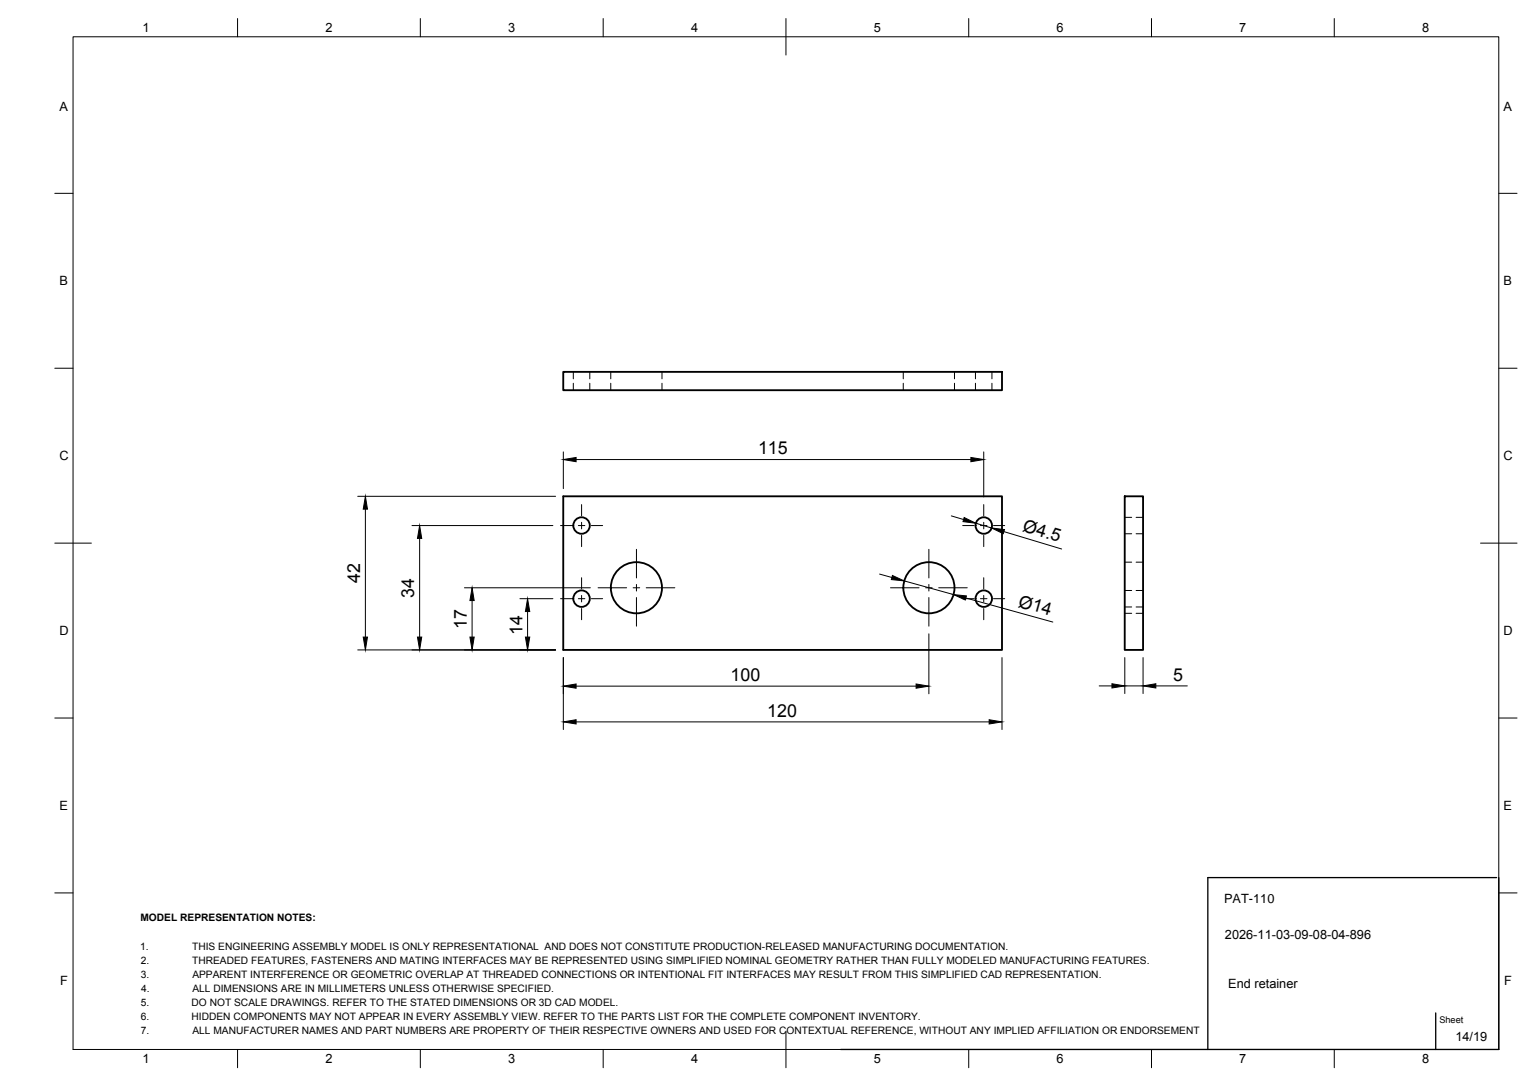
ISO-10303-21;
HEADER;
/* Generated by software containing ST-Developer
 * from STEP Tools, Inc. (www.steptools.com) 
 */

FILE_DESCRIPTION(
/* description */ ('Twin-shaft manual slide'),
/* implementation_level */ '2;1');

FILE_NAME(
/* name */ 'End retainer.step',
/* time_stamp */ '2026-10-27T18:38:08-07:00',
/* author */ (''),
/* organization */ (''),
/* preprocessor_version */ 'ST-DEVELOPER v20.2',
/* originating_system */ 'Autodesk Translation Framework v15.17.0.0',
/* authorisation */ '');

FILE_SCHEMA (('AUTOMOTIVE_DESIGN { 1 0 10303 214 3 1 1 }'));
ENDSEC;

DATA;
#10=MECHANICAL_DESIGN_GEOMETRIC_PRESENTATION_REPRESENTATION('',(#286),#6463);
#254=SHAPE_REPRESENTATION_RELATIONSHIP('SRR','None',#6574,#270);
#270=ADVANCED_BREP_SHAPE_REPRESENTATION('',(#301),#6457);
#286=STYLED_ITEM('',(#6726),#301);
#301=MANIFOLD_SOLID_BREP('Body1',#3649);
#382=FACE_BOUND('',#955,.T.);
#383=FACE_BOUND('',#956,.T.);
#384=FACE_BOUND('',#957,.T.);
#385=FACE_BOUND('',#958,.T.);
#386=FACE_BOUND('',#959,.T.);
#387=FACE_BOUND('',#960,.T.);
#388=FACE_BOUND('',#963,.T.);
#389=FACE_BOUND('',#964,.T.);
#390=FACE_BOUND('',#965,.T.);
#391=FACE_BOUND('',#966,.T.);
#392=FACE_BOUND('',#967,.T.);
#393=FACE_BOUND('',#968,.T.);
#483=PLANE('',#4115);
#484=PLANE('',#4116);
#485=PLANE('',#4117);
#486=PLANE('',#4118);
#487=PLANE('',#4119);
#488=PLANE('',#4120);
#662=FACE_OUTER_BOUND('',#947,.T.);
#663=FACE_OUTER_BOUND('',#948,.T.);
#664=FACE_OUTER_BOUND('',#949,.T.);
#665=FACE_OUTER_BOUND('',#950,.T.);
#666=FACE_OUTER_BOUND('',#951,.T.);
#667=FACE_OUTER_BOUND('',#952,.T.);
#668=FACE_OUTER_BOUND('',#953,.T.);
#669=FACE_OUTER_BOUND('',#954,.T.);
#670=FACE_OUTER_BOUND('',#961,.T.);
#671=FACE_OUTER_BOUND('',#962,.T.);
#672=FACE_OUTER_BOUND('',#969,.T.);
#673=FACE_OUTER_BOUND('',#970,.T.);
#947=EDGE_LOOP('',(#3090,#3091,#3092,#3093));
#948=EDGE_LOOP('',(#3094,#3095,#3096,#3097));
#949=EDGE_LOOP('',(#3098,#3099,#3100,#3101));
#950=EDGE_LOOP('',(#3102,#3103,#3104,#3105));
#951=EDGE_LOOP('',(#3106,#3107,#3108,#3109));
#952=EDGE_LOOP('',(#3110,#3111,#3112,#3113));
#953=EDGE_LOOP('',(#3114,#3115,#3116,#3117));
#954=EDGE_LOOP('',(#3118,#3119,#3120,#3121));
#955=EDGE_LOOP('',(#3122));
#956=EDGE_LOOP('',(#3123));
#957=EDGE_LOOP('',(#3124));
#958=EDGE_LOOP('',(#3125));
#959=EDGE_LOOP('',(#3126));
#960=EDGE_LOOP('',(#3127));
#961=EDGE_LOOP('',(#3128,#3129,#3130,#3131));
#962=EDGE_LOOP('',(#3132,#3133,#3134,#3135));
#963=EDGE_LOOP('',(#3136));
#964=EDGE_LOOP('',(#3137));
#965=EDGE_LOOP('',(#3138));
#966=EDGE_LOOP('',(#3139));
#967=EDGE_LOOP('',(#3140));
#968=EDGE_LOOP('',(#3141));
#969=EDGE_LOOP('',(#3142,#3143,#3144,#3145));
#970=EDGE_LOOP('',(#3146,#3147,#3148,#3149));
#1229=LINE('',#6074,#1515);
#1230=LINE('',#6080,#1516);
#1231=LINE('',#6086,#1517);
#1232=LINE('',#6092,#1518);
#1233=LINE('',#6098,#1519);
#1234=LINE('',#6104,#1520);
#1235=LINE('',#6109,#1521);
#1236=LINE('',#6111,#1522);
#1237=LINE('',#6113,#1523);
#1238=LINE('',#6114,#1524);
#1239=LINE('',#6117,#1525);
#1240=LINE('',#6119,#1526);
#1241=LINE('',#6120,#1527);
#1242=LINE('',#6123,#1528);
#1243=LINE('',#6125,#1529);
#1244=LINE('',#6126,#1530);
#1245=LINE('',#6128,#1531);
#1246=LINE('',#6129,#1532);
#1515=VECTOR('',#4987,0.225);
#1516=VECTOR('',#4994,0.225);
#1517=VECTOR('',#5001,0.225);
#1518=VECTOR('',#5008,0.225);
#1519=VECTOR('',#5015,0.7);
#1520=VECTOR('',#5022,0.7);
#1521=VECTOR('',#5027,1.);
#1522=VECTOR('',#5028,1.);
#1523=VECTOR('',#5029,1.);
#1524=VECTOR('',#5030,1.);
#1525=VECTOR('',#5033,1.);
#1526=VECTOR('',#5034,1.);
#1527=VECTOR('',#5035,1.);
#1528=VECTOR('',#5038,1.);
#1529=VECTOR('',#5039,1.);
#1530=VECTOR('',#5040,1.);
#1531=VECTOR('',#5043,1.);
#1532=VECTOR('',#5044,1.);
#1718=CIRCLE('',#4098,0.225);
#1719=CIRCLE('',#4099,0.225);
#1720=CIRCLE('',#4101,0.225);
#1721=CIRCLE('',#4102,0.225);
#1722=CIRCLE('',#4104,0.225);
#1723=CIRCLE('',#4105,0.225);
#1724=CIRCLE('',#4107,0.225);
#1725=CIRCLE('',#4108,0.225);
#1726=CIRCLE('',#4110,0.7);
#1727=CIRCLE('',#4111,0.7);
#1728=CIRCLE('',#4113,0.7);
#1729=CIRCLE('',#4114,0.7);
#1961=VERTEX_POINT('',#6071);
#1962=VERTEX_POINT('',#6073);
#1963=VERTEX_POINT('',#6077);
#1964=VERTEX_POINT('',#6079);
#1965=VERTEX_POINT('',#6083);
#1966=VERTEX_POINT('',#6085);
#1967=VERTEX_POINT('',#6089);
#1968=VERTEX_POINT('',#6091);
#1969=VERTEX_POINT('',#6095);
#1970=VERTEX_POINT('',#6097);
#1971=VERTEX_POINT('',#6101);
#1972=VERTEX_POINT('',#6103);
#1973=VERTEX_POINT('',#6107);
#1974=VERTEX_POINT('',#6108);
#1975=VERTEX_POINT('',#6110);
#1976=VERTEX_POINT('',#6112);
#1977=VERTEX_POINT('',#6116);
#1978=VERTEX_POINT('',#6118);
#1979=VERTEX_POINT('',#6122);
#1980=VERTEX_POINT('',#6124);
#2350=EDGE_CURVE('',#1961,#1961,#1718,.T.);
#2351=EDGE_CURVE('',#1961,#1962,#1229,.T.);
#2352=EDGE_CURVE('',#1962,#1962,#1719,.T.);
#2353=EDGE_CURVE('',#1963,#1963,#1720,.T.);
#2354=EDGE_CURVE('',#1963,#1964,#1230,.T.);
#2355=EDGE_CURVE('',#1964,#1964,#1721,.T.);
#2356=EDGE_CURVE('',#1965,#1965,#1722,.T.);
#2357=EDGE_CURVE('',#1965,#1966,#1231,.T.);
#2358=EDGE_CURVE('',#1966,#1966,#1723,.T.);
#2359=EDGE_CURVE('',#1967,#1967,#1724,.T.);
#2360=EDGE_CURVE('',#1967,#1968,#1232,.T.);
#2361=EDGE_CURVE('',#1968,#1968,#1725,.T.);
#2362=EDGE_CURVE('',#1969,#1969,#1726,.T.);
#2363=EDGE_CURVE('',#1969,#1970,#1233,.T.);
#2364=EDGE_CURVE('',#1970,#1970,#1727,.T.);
#2365=EDGE_CURVE('',#1971,#1971,#1728,.T.);
#2366=EDGE_CURVE('',#1971,#1972,#1234,.T.);
#2367=EDGE_CURVE('',#1972,#1972,#1729,.T.);
#2368=EDGE_CURVE('',#1973,#1974,#1235,.T.);
#2369=EDGE_CURVE('',#1974,#1975,#1236,.T.);
#2370=EDGE_CURVE('',#1976,#1975,#1237,.T.);
#2371=EDGE_CURVE('',#1973,#1976,#1238,.T.);
#2372=EDGE_CURVE('',#1977,#1973,#1239,.T.);
#2373=EDGE_CURVE('',#1978,#1976,#1240,.T.);
#2374=EDGE_CURVE('',#1977,#1978,#1241,.T.);
#2375=EDGE_CURVE('',#1979,#1977,#1242,.T.);
#2376=EDGE_CURVE('',#1980,#1978,#1243,.T.);
#2377=EDGE_CURVE('',#1979,#1980,#1244,.T.);
#2378=EDGE_CURVE('',#1974,#1979,#1245,.T.);
#2379=EDGE_CURVE('',#1975,#1980,#1246,.T.);
#3090=ORIENTED_EDGE('',*,*,#2350,.F.);
#3091=ORIENTED_EDGE('',*,*,#2351,.T.);
#3092=ORIENTED_EDGE('',*,*,#2352,.F.);
#3093=ORIENTED_EDGE('',*,*,#2351,.F.);
#3094=ORIENTED_EDGE('',*,*,#2353,.F.);
#3095=ORIENTED_EDGE('',*,*,#2354,.T.);
#3096=ORIENTED_EDGE('',*,*,#2355,.F.);
#3097=ORIENTED_EDGE('',*,*,#2354,.F.);
#3098=ORIENTED_EDGE('',*,*,#2356,.F.);
#3099=ORIENTED_EDGE('',*,*,#2357,.T.);
#3100=ORIENTED_EDGE('',*,*,#2358,.F.);
#3101=ORIENTED_EDGE('',*,*,#2357,.F.);
#3102=ORIENTED_EDGE('',*,*,#2359,.F.);
#3103=ORIENTED_EDGE('',*,*,#2360,.T.);
#3104=ORIENTED_EDGE('',*,*,#2361,.F.);
#3105=ORIENTED_EDGE('',*,*,#2360,.F.);
#3106=ORIENTED_EDGE('',*,*,#2362,.F.);
#3107=ORIENTED_EDGE('',*,*,#2363,.T.);
#3108=ORIENTED_EDGE('',*,*,#2364,.F.);
#3109=ORIENTED_EDGE('',*,*,#2363,.F.);
#3110=ORIENTED_EDGE('',*,*,#2365,.F.);
#3111=ORIENTED_EDGE('',*,*,#2366,.T.);
#3112=ORIENTED_EDGE('',*,*,#2367,.F.);
#3113=ORIENTED_EDGE('',*,*,#2366,.F.);
#3114=ORIENTED_EDGE('',*,*,#2368,.T.);
#3115=ORIENTED_EDGE('',*,*,#2369,.T.);
#3116=ORIENTED_EDGE('',*,*,#2370,.F.);
#3117=ORIENTED_EDGE('',*,*,#2371,.F.);
#3118=ORIENTED_EDGE('',*,*,#2372,.T.);
#3119=ORIENTED_EDGE('',*,*,#2371,.T.);
#3120=ORIENTED_EDGE('',*,*,#2373,.F.);
#3121=ORIENTED_EDGE('',*,*,#2374,.F.);
#3122=ORIENTED_EDGE('',*,*,#2367,.T.);
#3123=ORIENTED_EDGE('',*,*,#2364,.T.);
#3124=ORIENTED_EDGE('',*,*,#2361,.T.);
#3125=ORIENTED_EDGE('',*,*,#2358,.T.);
#3126=ORIENTED_EDGE('',*,*,#2355,.T.);
#3127=ORIENTED_EDGE('',*,*,#2352,.T.);
#3128=ORIENTED_EDGE('',*,*,#2375,.T.);
#3129=ORIENTED_EDGE('',*,*,#2374,.T.);
#3130=ORIENTED_EDGE('',*,*,#2376,.F.);
#3131=ORIENTED_EDGE('',*,*,#2377,.F.);
#3132=ORIENTED_EDGE('',*,*,#2378,.T.);
#3133=ORIENTED_EDGE('',*,*,#2377,.T.);
#3134=ORIENTED_EDGE('',*,*,#2379,.F.);
#3135=ORIENTED_EDGE('',*,*,#2369,.F.);
#3136=ORIENTED_EDGE('',*,*,#2365,.T.);
#3137=ORIENTED_EDGE('',*,*,#2362,.T.);
#3138=ORIENTED_EDGE('',*,*,#2359,.T.);
#3139=ORIENTED_EDGE('',*,*,#2356,.T.);
#3140=ORIENTED_EDGE('',*,*,#2353,.T.);
#3141=ORIENTED_EDGE('',*,*,#2350,.T.);
#3142=ORIENTED_EDGE('',*,*,#2379,.T.);
#3143=ORIENTED_EDGE('',*,*,#2376,.T.);
#3144=ORIENTED_EDGE('',*,*,#2373,.T.);
#3145=ORIENTED_EDGE('',*,*,#2370,.T.);
#3146=ORIENTED_EDGE('',*,*,#2378,.F.);
#3147=ORIENTED_EDGE('',*,*,#2368,.F.);
#3148=ORIENTED_EDGE('',*,*,#2372,.F.);
#3149=ORIENTED_EDGE('',*,*,#2375,.F.);
#3415=CYLINDRICAL_SURFACE('',#4097,0.225);
#3416=CYLINDRICAL_SURFACE('',#4100,0.225);
#3417=CYLINDRICAL_SURFACE('',#4103,0.225);
#3418=CYLINDRICAL_SURFACE('',#4106,0.225);
#3419=CYLINDRICAL_SURFACE('',#4109,0.7);
#3420=CYLINDRICAL_SURFACE('',#4112,0.7);
#3567=ADVANCED_FACE('',(#662),#3415,.F.);
#3568=ADVANCED_FACE('',(#663),#3416,.F.);
#3569=ADVANCED_FACE('',(#664),#3417,.F.);
#3570=ADVANCED_FACE('',(#665),#3418,.F.);
#3571=ADVANCED_FACE('',(#666),#3419,.F.);
#3572=ADVANCED_FACE('',(#667),#3420,.F.);
#3573=ADVANCED_FACE('',(#668),#483,.T.);
#3574=ADVANCED_FACE('',(#669,#382,#383,#384,#385,#386,#387),#484,.T.);
#3575=ADVANCED_FACE('',(#670),#485,.T.);
#3576=ADVANCED_FACE('',(#671,#388,#389,#390,#391,#392,#393),#486,.T.);
#3577=ADVANCED_FACE('',(#672),#487,.T.);
#3578=ADVANCED_FACE('',(#673),#488,.F.);
#3649=CLOSED_SHELL('',(#3567,#3568,#3569,#3570,#3571,#3572,#3573,#3574,
#3575,#3576,#3577,#3578));
#4096=AXIS2_PLACEMENT_3D('',#6069,#4981,#4982);
#4097=AXIS2_PLACEMENT_3D('',#6070,#4983,#4984);
#4098=AXIS2_PLACEMENT_3D('',#6072,#4985,#4986);
#4099=AXIS2_PLACEMENT_3D('',#6075,#4988,#4989);
#4100=AXIS2_PLACEMENT_3D('',#6076,#4990,#4991);
#4101=AXIS2_PLACEMENT_3D('',#6078,#4992,#4993);
#4102=AXIS2_PLACEMENT_3D('',#6081,#4995,#4996);
#4103=AXIS2_PLACEMENT_3D('',#6082,#4997,#4998);
#4104=AXIS2_PLACEMENT_3D('',#6084,#4999,#5000);
#4105=AXIS2_PLACEMENT_3D('',#6087,#5002,#5003);
#4106=AXIS2_PLACEMENT_3D('',#6088,#5004,#5005);
#4107=AXIS2_PLACEMENT_3D('',#6090,#5006,#5007);
#4108=AXIS2_PLACEMENT_3D('',#6093,#5009,#5010);
#4109=AXIS2_PLACEMENT_3D('',#6094,#5011,#5012);
#4110=AXIS2_PLACEMENT_3D('',#6096,#5013,#5014);
#4111=AXIS2_PLACEMENT_3D('',#6099,#5016,#5017);
#4112=AXIS2_PLACEMENT_3D('',#6100,#5018,#5019);
#4113=AXIS2_PLACEMENT_3D('',#6102,#5020,#5021);
#4114=AXIS2_PLACEMENT_3D('',#6105,#5023,#5024);
#4115=AXIS2_PLACEMENT_3D('',#6106,#5025,#5026);
#4116=AXIS2_PLACEMENT_3D('',#6115,#5031,#5032);
#4117=AXIS2_PLACEMENT_3D('',#6121,#5036,#5037);
#4118=AXIS2_PLACEMENT_3D('',#6127,#5041,#5042);
#4119=AXIS2_PLACEMENT_3D('',#6130,#5045,#5046);
#4120=AXIS2_PLACEMENT_3D('',#6131,#5047,#5048);
#4981=DIRECTION('axis',(0.,0.,1.));
#4982=DIRECTION('refdir',(1.,0.,0.));
#4983=DIRECTION('center_axis',(1.,0.,0.));
#4984=DIRECTION('ref_axis',(0.,0.,-1.));
#4985=DIRECTION('center_axis',(1.,0.,0.));
#4986=DIRECTION('ref_axis',(0.,0.,-1.));
#4987=DIRECTION('',(1.,0.,0.));
#4988=DIRECTION('center_axis',(-1.,0.,0.));
#4989=DIRECTION('ref_axis',(0.,0.,-1.));
#4990=DIRECTION('center_axis',(1.,0.,0.));
#4991=DIRECTION('ref_axis',(0.,0.,-1.));
#4992=DIRECTION('center_axis',(1.,0.,0.));
#4993=DIRECTION('ref_axis',(0.,0.,-1.));
#4994=DIRECTION('',(1.,0.,0.));
#4995=DIRECTION('center_axis',(-1.,0.,0.));
#4996=DIRECTION('ref_axis',(0.,0.,-1.));
#4997=DIRECTION('center_axis',(1.,0.,0.));
#4998=DIRECTION('ref_axis',(0.,0.,-1.));
#4999=DIRECTION('center_axis',(1.,0.,0.));
#5000=DIRECTION('ref_axis',(0.,0.,-1.));
#5001=DIRECTION('',(1.,0.,0.));
#5002=DIRECTION('center_axis',(-1.,0.,0.));
#5003=DIRECTION('ref_axis',(0.,0.,-1.));
#5004=DIRECTION('center_axis',(1.,0.,0.));
#5005=DIRECTION('ref_axis',(0.,0.,-1.));
#5006=DIRECTION('center_axis',(1.,0.,0.));
#5007=DIRECTION('ref_axis',(0.,0.,-1.));
#5008=DIRECTION('',(1.,0.,0.));
#5009=DIRECTION('center_axis',(-1.,0.,0.));
#5010=DIRECTION('ref_axis',(0.,0.,-1.));
#5011=DIRECTION('center_axis',(1.,0.,0.));
#5012=DIRECTION('ref_axis',(0.,0.,-1.));
#5013=DIRECTION('center_axis',(1.,0.,0.));
#5014=DIRECTION('ref_axis',(0.,0.,-1.));
#5015=DIRECTION('',(1.,0.,0.));
#5016=DIRECTION('center_axis',(-1.,0.,0.));
#5017=DIRECTION('ref_axis',(0.,0.,-1.));
#5018=DIRECTION('center_axis',(1.,0.,0.));
#5019=DIRECTION('ref_axis',(0.,0.,-1.));
#5020=DIRECTION('center_axis',(1.,0.,0.));
#5021=DIRECTION('ref_axis',(0.,0.,-1.));
#5022=DIRECTION('',(1.,0.,0.));
#5023=DIRECTION('center_axis',(-1.,0.,0.));
#5024=DIRECTION('ref_axis',(0.,0.,-1.));
#5025=DIRECTION('center_axis',(0.,1.,0.));
#5026=DIRECTION('ref_axis',(-1.,0.,0.));
#5027=DIRECTION('',(-1.,0.,0.));
#5028=DIRECTION('',(0.,0.,1.));
#5029=DIRECTION('',(-1.,0.,0.));
#5030=DIRECTION('',(0.,0.,1.));
#5031=DIRECTION('center_axis',(1.,0.,0.));
#5032=DIRECTION('ref_axis',(0.,1.,0.));
#5033=DIRECTION('',(0.,1.,0.));
#5034=DIRECTION('',(0.,1.,0.));
#5035=DIRECTION('',(0.,0.,1.));
#5036=DIRECTION('center_axis',(0.,-1.,0.));
#5037=DIRECTION('ref_axis',(1.,0.,0.));
#5038=DIRECTION('',(1.,0.,0.));
#5039=DIRECTION('',(1.,0.,0.));
#5040=DIRECTION('',(0.,0.,1.));
#5041=DIRECTION('center_axis',(-1.,0.,0.));
#5042=DIRECTION('ref_axis',(0.,-1.,0.));
#5043=DIRECTION('',(0.,-1.,0.));
#5044=DIRECTION('',(0.,-1.,0.));
#5045=DIRECTION('center_axis',(0.,0.,1.));
#5046=DIRECTION('ref_axis',(1.,0.,0.));
#5047=DIRECTION('center_axis',(0.,0.,1.));
#5048=DIRECTION('ref_axis',(1.,0.,0.));
#6069=CARTESIAN_POINT('',(0.,0.,0.));
#6070=CARTESIAN_POINT('Origin',(9.9,5.5,3.));
#6071=CARTESIAN_POINT('',(10.,5.5,3.225));
#6072=CARTESIAN_POINT('Origin',(10.,5.5,3.));
#6073=CARTESIAN_POINT('',(10.5,5.5,3.225));
#6074=CARTESIAN_POINT('',(9.9,5.5,3.225));
#6075=CARTESIAN_POINT('Origin',(10.5,5.5,3.));
#6076=CARTESIAN_POINT('Origin',(9.9,-5.5,5.));
#6077=CARTESIAN_POINT('',(10.,-5.5,5.225));
#6078=CARTESIAN_POINT('Origin',(10.,-5.5,5.));
#6079=CARTESIAN_POINT('',(10.5,-5.5,5.225));
#6080=CARTESIAN_POINT('',(9.9,-5.5,5.225));
#6081=CARTESIAN_POINT('Origin',(10.5,-5.5,5.));
#6082=CARTESIAN_POINT('Origin',(9.9,-5.5,3.));
#6083=CARTESIAN_POINT('',(10.,-5.5,3.225));
#6084=CARTESIAN_POINT('Origin',(10.,-5.5,3.));
#6085=CARTESIAN_POINT('',(10.5,-5.5,3.225));
#6086=CARTESIAN_POINT('',(9.9,-5.5,3.225));
#6087=CARTESIAN_POINT('Origin',(10.5,-5.5,3.));
#6088=CARTESIAN_POINT('Origin',(9.9,5.5,5.));
#6089=CARTESIAN_POINT('',(10.,5.5,5.225));
#6090=CARTESIAN_POINT('Origin',(10.,5.5,5.));
#6091=CARTESIAN_POINT('',(10.5,5.5,5.225));
#6092=CARTESIAN_POINT('',(9.9,5.5,5.225));
#6093=CARTESIAN_POINT('Origin',(10.5,5.5,5.));
#6094=CARTESIAN_POINT('Origin',(9.9,-4.,3.3));
#6095=CARTESIAN_POINT('',(10.,-4.,4.));
#6096=CARTESIAN_POINT('Origin',(10.,-4.,3.3));
#6097=CARTESIAN_POINT('',(10.5,-4.,4.));
#6098=CARTESIAN_POINT('',(9.9,-4.,4.));
#6099=CARTESIAN_POINT('Origin',(10.5,-4.,3.3));
#6100=CARTESIAN_POINT('Origin',(9.9,4.,3.3));
#6101=CARTESIAN_POINT('',(10.,4.,4.));
#6102=CARTESIAN_POINT('Origin',(10.,4.,3.3));
#6103=CARTESIAN_POINT('',(10.5,4.,4.));
#6104=CARTESIAN_POINT('',(9.9,4.,4.));
#6105=CARTESIAN_POINT('Origin',(10.5,4.,3.3));
#6106=CARTESIAN_POINT('Origin',(10.5,6.,1.6));
#6107=CARTESIAN_POINT('',(10.5,6.,1.6));
#6108=CARTESIAN_POINT('',(10.,6.,1.6));
#6109=CARTESIAN_POINT('',(10.5,6.,1.6));
#6110=CARTESIAN_POINT('',(10.,6.,5.8));
#6111=CARTESIAN_POINT('',(10.,6.,1.6));
#6112=CARTESIAN_POINT('',(10.5,6.,5.8));
#6113=CARTESIAN_POINT('',(10.5,6.,5.8));
#6114=CARTESIAN_POINT('',(10.5,6.,1.6));
#6115=CARTESIAN_POINT('Origin',(10.5,-6.,1.6));
#6116=CARTESIAN_POINT('',(10.5,-6.,1.6));
#6117=CARTESIAN_POINT('',(10.5,-6.,1.6));
#6118=CARTESIAN_POINT('',(10.5,-6.,5.8));
#6119=CARTESIAN_POINT('',(10.5,-6.,5.8));
#6120=CARTESIAN_POINT('',(10.5,-6.,1.6));
#6121=CARTESIAN_POINT('Origin',(10.,-6.,1.6));
#6122=CARTESIAN_POINT('',(10.,-6.,1.6));
#6123=CARTESIAN_POINT('',(10.,-6.,1.6));
#6124=CARTESIAN_POINT('',(10.,-6.,5.8));
#6125=CARTESIAN_POINT('',(10.,-6.,5.8));
#6126=CARTESIAN_POINT('',(10.,-6.,1.6));
#6127=CARTESIAN_POINT('Origin',(10.,6.,1.6));
#6128=CARTESIAN_POINT('',(10.,6.,1.6));
#6129=CARTESIAN_POINT('',(10.,6.,5.8));
#6130=CARTESIAN_POINT('Origin',(10.25,0.,5.8));
#6131=CARTESIAN_POINT('Origin',(10.25,0.,1.6));
#6436=UNCERTAINTY_MEASURE_WITH_UNIT(LENGTH_MEASURE(0.001),#6464,
'DISTANCE_ACCURACY_VALUE',
'Maximum model space distance between geometric entities at asserted c
onnectivities');
#6442=UNCERTAINTY_MEASURE_WITH_UNIT(LENGTH_MEASURE(0.001),#6464,
'DISTANCE_ACCURACY_VALUE',
'Maximum model space distance between geometric entities at asserted c
onnectivities');
#6457=(
GEOMETRIC_REPRESENTATION_CONTEXT(3)
GLOBAL_UNCERTAINTY_ASSIGNED_CONTEXT((#6436))
GLOBAL_UNIT_ASSIGNED_CONTEXT((#6464,#6466,#6467))
REPRESENTATION_CONTEXT('','3D')
);
#6463=(
GEOMETRIC_REPRESENTATION_CONTEXT(3)
GLOBAL_UNCERTAINTY_ASSIGNED_CONTEXT((#6442))
GLOBAL_UNIT_ASSIGNED_CONTEXT((#6464,#6466,#6467))
REPRESENTATION_CONTEXT('','3D')
);
#6464=(
LENGTH_UNIT()
NAMED_UNIT(*)
SI_UNIT(.CENTI.,.METRE.)
);
#6466=(
NAMED_UNIT(*)
PLANE_ANGLE_UNIT()
SI_UNIT($,.RADIAN.)
);
#6467=(
NAMED_UNIT(*)
SI_UNIT($,.STERADIAN.)
SOLID_ANGLE_UNIT()
);
#6482=SHAPE_DEFINITION_REPRESENTATION(#6504,#6574);
#6504=PRODUCT_DEFINITION_SHAPE('',$,#6595);
#6574=SHAPE_REPRESENTATION('',(#4096),#6457);
#6580=PRODUCT_DEFINITION_CONTEXT('part definition',#6642,'design');
#6595=PRODUCT_DEFINITION('End retainer','End retainer',#6615,#6580);
#6615=PRODUCT_DEFINITION_FORMATION('',$,#6658);
#6642=APPLICATION_CONTEXT(
'Core Data for Automotive Mechanical Design Process');
#6643=PRODUCT_CONTEXT('part definition',#6642,'mechanical');
#6658=PRODUCT('End retainer','End retainer','End retainer',(#6643));
#6720=COLOUR_RGB('Light Blue',0.38,0.62,0.78);
#6721=FILL_AREA_STYLE_COLOUR('',#6720);
#6722=FILL_AREA_STYLE('',(#6721));
#6723=SURFACE_STYLE_FILL_AREA(#6722);
#6724=SURFACE_SIDE_STYLE('',(#6723));
#6725=SURFACE_STYLE_USAGE(.BOTH.,#6724);
#6726=PRESENTATION_STYLE_ASSIGNMENT((#6725));
ENDSEC;
END-ISO-10303-21;
